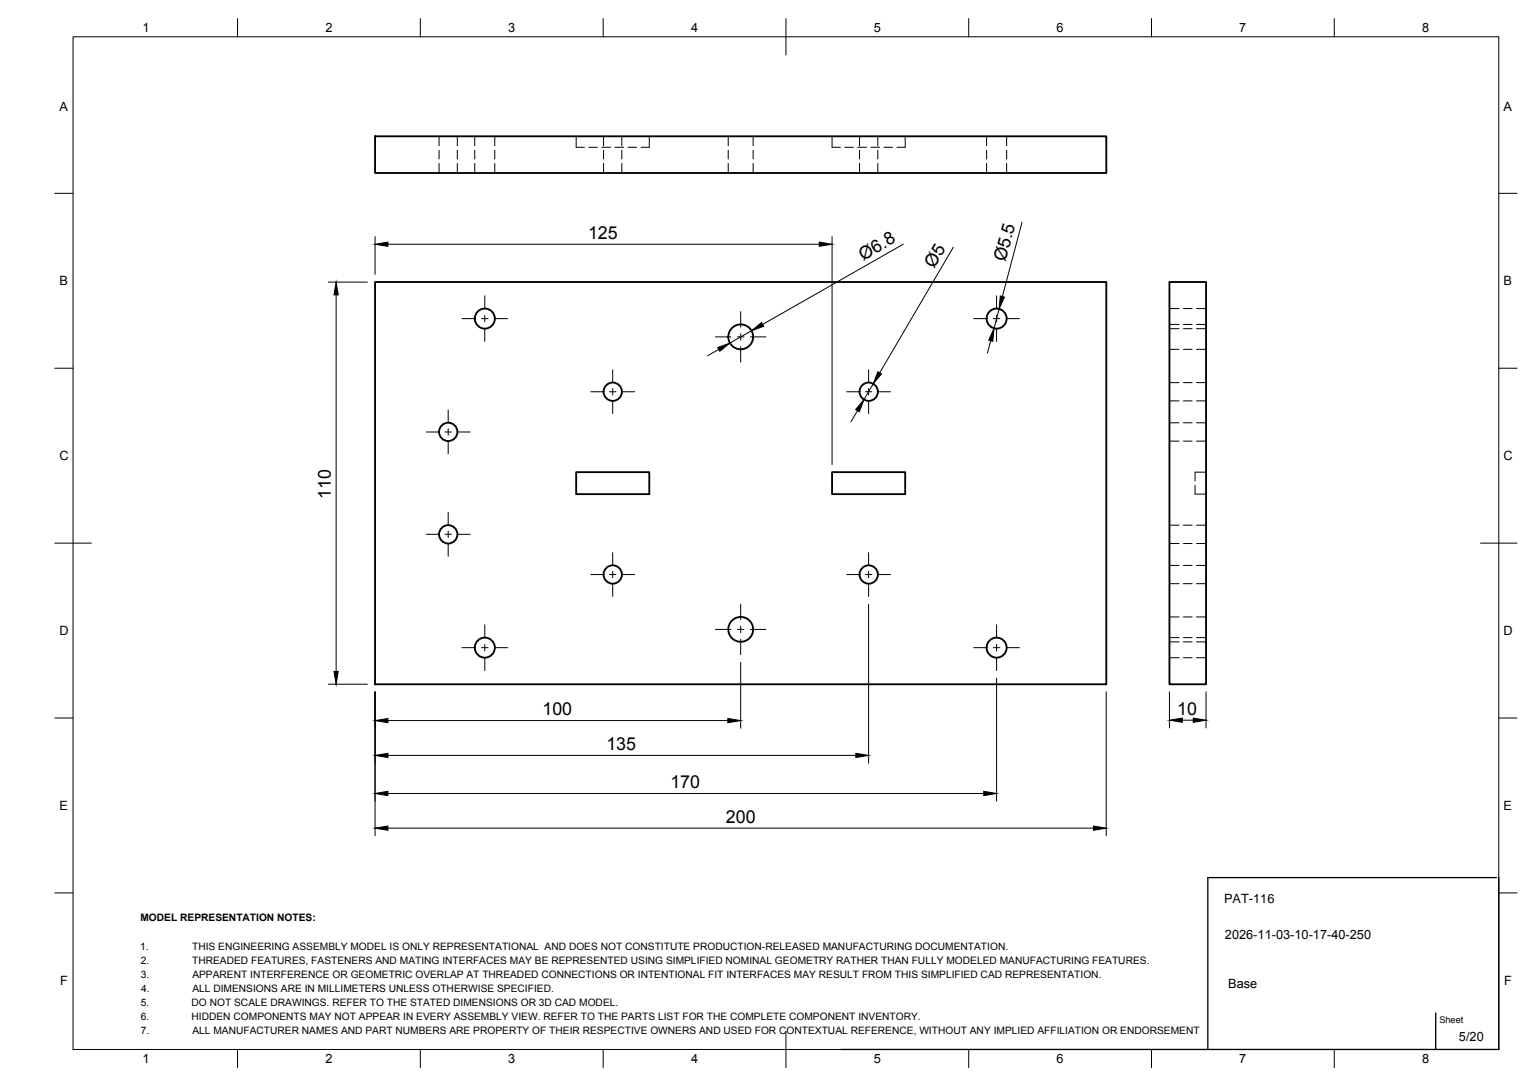
ISO-10303-21;
HEADER;
/* Generated by software containing ST-Developer
 * from STEP Tools, Inc. (www.steptools.com) 
 */

FILE_DESCRIPTION(
/* description */ ('V-block with clamp strap'),
/* implementation_level */ '2;1');

FILE_NAME(
/* name */ 'Base.step',
/* time_stamp */ '2026-10-27T10:50:53-07:00',
/* author */ (''),
/* organization */ (''),
/* preprocessor_version */ 'ST-DEVELOPER v20.2',
/* originating_system */ 'Autodesk Translation Framework v15.17.0.0',
/* authorisation */ '');

FILE_SCHEMA (('AUTOMOTIVE_DESIGN { 1 0 10303 214 3 1 1 }'));
ENDSEC;

DATA;
#10=MECHANICAL_DESIGN_GEOMETRIC_PRESENTATION_REPRESENTATION('',(#266),#7344);
#224=SHAPE_REPRESENTATION_RELATIONSHIP('SRR','None',#7442,#245);
#245=ADVANCED_BREP_SHAPE_REPRESENTATION('',(#287),#7321);
#266=STYLED_ITEM('',(#7610),#287);
#287=MANIFOLD_SOLID_BREP('Body1',#4148);
#305=FACE_BOUND('',#829,.T.);
#306=FACE_BOUND('',#830,.T.);
#307=FACE_BOUND('',#831,.T.);
#308=FACE_BOUND('',#832,.T.);
#309=FACE_BOUND('',#833,.T.);
#310=FACE_BOUND('',#834,.T.);
#311=FACE_BOUND('',#835,.T.);
#312=FACE_BOUND('',#836,.T.);
#313=FACE_BOUND('',#837,.T.);
#314=FACE_BOUND('',#838,.T.);
#315=FACE_BOUND('',#839,.T.);
#316=FACE_BOUND('',#840,.T.);
#317=FACE_BOUND('',#841,.T.);
#318=FACE_BOUND('',#842,.T.);
#319=FACE_BOUND('',#844,.T.);
#320=FACE_BOUND('',#845,.T.);
#321=FACE_BOUND('',#846,.T.);
#322=FACE_BOUND('',#847,.T.);
#323=FACE_BOUND('',#848,.T.);
#324=FACE_BOUND('',#849,.T.);
#325=FACE_BOUND('',#850,.T.);
#326=FACE_BOUND('',#851,.T.);
#327=FACE_BOUND('',#852,.T.);
#328=FACE_BOUND('',#853,.T.);
#329=FACE_BOUND('',#854,.T.);
#330=FACE_BOUND('',#855,.T.);
#376=CIRCLE('',#4418,0.274999999999999);
#377=CIRCLE('',#4419,0.274999999999999);
#378=CIRCLE('',#4421,0.275);
#379=CIRCLE('',#4422,0.275);
#380=CIRCLE('',#4424,0.275);
#381=CIRCLE('',#4425,0.275);
#382=CIRCLE('',#4427,0.274999999999999);
#383=CIRCLE('',#4428,0.274999999999999);
#384=CIRCLE('',#4430,0.34);
#385=CIRCLE('',#4431,0.34);
#386=CIRCLE('',#4433,0.34);
#387=CIRCLE('',#4434,0.34);
#388=CIRCLE('',#4436,0.25);
#389=CIRCLE('',#4437,0.25);
#390=CIRCLE('',#4439,0.25);
#391=CIRCLE('',#4440,0.25);
#392=CIRCLE('',#4442,0.25);
#393=CIRCLE('',#4443,0.25);
#394=CIRCLE('',#4445,0.25);
#395=CIRCLE('',#4446,0.25);
#396=CIRCLE('',#4448,0.25);
#397=CIRCLE('',#4449,0.25);
#398=CIRCLE('',#4451,0.25);
#399=CIRCLE('',#4452,0.25);
#505=CYLINDRICAL_SURFACE('',#4417,0.274999999999999);
#506=CYLINDRICAL_SURFACE('',#4420,0.275);
#507=CYLINDRICAL_SURFACE('',#4423,0.275);
#508=CYLINDRICAL_SURFACE('',#4426,0.274999999999999);
#509=CYLINDRICAL_SURFACE('',#4429,0.34);
#510=CYLINDRICAL_SURFACE('',#4432,0.34);
#511=CYLINDRICAL_SURFACE('',#4435,0.25);
#512=CYLINDRICAL_SURFACE('',#4438,0.25);
#513=CYLINDRICAL_SURFACE('',#4441,0.25);
#514=CYLINDRICAL_SURFACE('',#4444,0.25);
#515=CYLINDRICAL_SURFACE('',#4447,0.25);
#516=CYLINDRICAL_SURFACE('',#4450,0.25);
#562=FACE_OUTER_BOUND('',#802,.T.);
#563=FACE_OUTER_BOUND('',#803,.T.);
#564=FACE_OUTER_BOUND('',#804,.T.);
#565=FACE_OUTER_BOUND('',#805,.T.);
#566=FACE_OUTER_BOUND('',#806,.T.);
#567=FACE_OUTER_BOUND('',#807,.T.);
#568=FACE_OUTER_BOUND('',#808,.T.);
#569=FACE_OUTER_BOUND('',#809,.T.);
#570=FACE_OUTER_BOUND('',#810,.T.);
#571=FACE_OUTER_BOUND('',#811,.T.);
#572=FACE_OUTER_BOUND('',#812,.T.);
#573=FACE_OUTER_BOUND('',#813,.T.);
#574=FACE_OUTER_BOUND('',#814,.T.);
#575=FACE_OUTER_BOUND('',#815,.T.);
#576=FACE_OUTER_BOUND('',#816,.T.);
#577=FACE_OUTER_BOUND('',#817,.T.);
#578=FACE_OUTER_BOUND('',#818,.T.);
#579=FACE_OUTER_BOUND('',#819,.T.);
#580=FACE_OUTER_BOUND('',#820,.T.);
#581=FACE_OUTER_BOUND('',#821,.T.);
#582=FACE_OUTER_BOUND('',#822,.T.);
#583=FACE_OUTER_BOUND('',#823,.T.);
#584=FACE_OUTER_BOUND('',#824,.T.);
#585=FACE_OUTER_BOUND('',#825,.T.);
#586=FACE_OUTER_BOUND('',#826,.T.);
#587=FACE_OUTER_BOUND('',#827,.T.);
#588=FACE_OUTER_BOUND('',#828,.T.);
#589=FACE_OUTER_BOUND('',#843,.T.);
#802=EDGE_LOOP('',(#2696,#2697,#2698,#2699));
#803=EDGE_LOOP('',(#2700,#2701,#2702,#2703));
#804=EDGE_LOOP('',(#2704,#2705,#2706,#2707));
#805=EDGE_LOOP('',(#2708,#2709,#2710,#2711));
#806=EDGE_LOOP('',(#2712,#2713,#2714,#2715));
#807=EDGE_LOOP('',(#2716,#2717,#2718,#2719));
#808=EDGE_LOOP('',(#2720,#2721,#2722,#2723));
#809=EDGE_LOOP('',(#2724,#2725,#2726,#2727));
#810=EDGE_LOOP('',(#2728,#2729,#2730,#2731));
#811=EDGE_LOOP('',(#2732,#2733,#2734,#2735));
#812=EDGE_LOOP('',(#2736,#2737,#2738,#2739));
#813=EDGE_LOOP('',(#2740,#2741,#2742,#2743));
#814=EDGE_LOOP('',(#2744,#2745,#2746,#2747));
#815=EDGE_LOOP('',(#2748,#2749,#2750,#2751));
#816=EDGE_LOOP('',(#2752,#2753,#2754,#2755));
#817=EDGE_LOOP('',(#2756,#2757,#2758,#2759));
#818=EDGE_LOOP('',(#2760,#2761,#2762,#2763));
#819=EDGE_LOOP('',(#2764,#2765,#2766,#2767));
#820=EDGE_LOOP('',(#2768,#2769,#2770,#2771));
#821=EDGE_LOOP('',(#2772,#2773,#2774,#2775));
#822=EDGE_LOOP('',(#2776,#2777,#2778,#2779));
#823=EDGE_LOOP('',(#2780,#2781,#2782,#2783));
#824=EDGE_LOOP('',(#2784,#2785,#2786,#2787));
#825=EDGE_LOOP('',(#2788,#2789,#2790,#2791));
#826=EDGE_LOOP('',(#2792,#2793,#2794,#2795));
#827=EDGE_LOOP('',(#2796,#2797,#2798,#2799));
#828=EDGE_LOOP('',(#2800,#2801,#2802,#2803));
#829=EDGE_LOOP('',(#2804,#2805,#2806,#2807));
#830=EDGE_LOOP('',(#2808));
#831=EDGE_LOOP('',(#2809));
#832=EDGE_LOOP('',(#2810));
#833=EDGE_LOOP('',(#2811));
#834=EDGE_LOOP('',(#2812));
#835=EDGE_LOOP('',(#2813));
#836=EDGE_LOOP('',(#2814));
#837=EDGE_LOOP('',(#2815));
#838=EDGE_LOOP('',(#2816));
#839=EDGE_LOOP('',(#2817));
#840=EDGE_LOOP('',(#2818));
#841=EDGE_LOOP('',(#2819));
#842=EDGE_LOOP('',(#2820,#2821,#2822,#2823));
#843=EDGE_LOOP('',(#2824,#2825,#2826,#2827));
#844=EDGE_LOOP('',(#2828));
#845=EDGE_LOOP('',(#2829));
#846=EDGE_LOOP('',(#2830));
#847=EDGE_LOOP('',(#2831));
#848=EDGE_LOOP('',(#2832));
#849=EDGE_LOOP('',(#2833));
#850=EDGE_LOOP('',(#2834));
#851=EDGE_LOOP('',(#2835));
#852=EDGE_LOOP('',(#2836));
#853=EDGE_LOOP('',(#2837));
#854=EDGE_LOOP('',(#2838));
#855=EDGE_LOOP('',(#2839));
#1113=LINE('',#6092,#1478);
#1114=LINE('',#6094,#1479);
#1115=LINE('',#6096,#1480);
#1116=LINE('',#6097,#1481);
#1117=LINE('',#6100,#1482);
#1118=LINE('',#6102,#1483);
#1119=LINE('',#6103,#1484);
#1120=LINE('',#6106,#1485);
#1121=LINE('',#6108,#1486);
#1122=LINE('',#6109,#1487);
#1123=LINE('',#6111,#1488);
#1124=LINE('',#6112,#1489);
#1125=LINE('',#6117,#1490);
#1126=LINE('',#6119,#1491);
#1127=LINE('',#6121,#1492);
#1128=LINE('',#6122,#1493);
#1129=LINE('',#6125,#1494);
#1130=LINE('',#6127,#1495);
#1131=LINE('',#6128,#1496);
#1132=LINE('',#6131,#1497);
#1133=LINE('',#6133,#1498);
#1134=LINE('',#6134,#1499);
#1135=LINE('',#6136,#1500);
#1136=LINE('',#6137,#1501);
#1137=LINE('',#6143,#1502);
#1138=LINE('',#6149,#1503);
#1139=LINE('',#6155,#1504);
#1140=LINE('',#6161,#1505);
#1141=LINE('',#6167,#1506);
#1142=LINE('',#6173,#1507);
#1143=LINE('',#6179,#1508);
#1144=LINE('',#6185,#1509);
#1145=LINE('',#6191,#1510);
#1146=LINE('',#6197,#1511);
#1147=LINE('',#6203,#1512);
#1148=LINE('',#6209,#1513);
#1149=LINE('',#6214,#1514);
#1150=LINE('',#6216,#1515);
#1151=LINE('',#6218,#1516);
#1152=LINE('',#6219,#1517);
#1153=LINE('',#6222,#1518);
#1154=LINE('',#6224,#1519);
#1155=LINE('',#6225,#1520);
#1156=LINE('',#6228,#1521);
#1157=LINE('',#6230,#1522);
#1158=LINE('',#6231,#1523);
#1159=LINE('',#6233,#1524);
#1160=LINE('',#6234,#1525);
#1478=VECTOR('',#4851,1.);
#1479=VECTOR('',#4852,1.);
#1480=VECTOR('',#4853,1.);
#1481=VECTOR('',#4854,1.);
#1482=VECTOR('',#4857,1.);
#1483=VECTOR('',#4858,1.);
#1484=VECTOR('',#4859,1.);
#1485=VECTOR('',#4862,1.);
#1486=VECTOR('',#4863,1.);
#1487=VECTOR('',#4864,1.);
#1488=VECTOR('',#4867,1.);
#1489=VECTOR('',#4868,1.);
#1490=VECTOR('',#4873,1.);
#1491=VECTOR('',#4874,1.);
#1492=VECTOR('',#4875,1.);
#1493=VECTOR('',#4876,1.);
#1494=VECTOR('',#4879,1.);
#1495=VECTOR('',#4880,1.);
#1496=VECTOR('',#4881,1.);
#1497=VECTOR('',#4884,1.);
#1498=VECTOR('',#4885,1.);
#1499=VECTOR('',#4886,1.);
#1500=VECTOR('',#4889,1.);
#1501=VECTOR('',#4890,1.);
#1502=VECTOR('',#4897,0.274999999999999);
#1503=VECTOR('',#4904,0.275);
#1504=VECTOR('',#4911,0.275);
#1505=VECTOR('',#4918,0.274999999999999);
#1506=VECTOR('',#4925,0.34);
#1507=VECTOR('',#4932,0.34);
#1508=VECTOR('',#4939,0.25);
#1509=VECTOR('',#4946,0.25);
#1510=VECTOR('',#4953,0.25);
#1511=VECTOR('',#4960,0.25);
#1512=VECTOR('',#4967,0.25);
#1513=VECTOR('',#4974,0.25);
#1514=VECTOR('',#4979,1.);
#1515=VECTOR('',#4980,1.);
#1516=VECTOR('',#4981,1.);
#1517=VECTOR('',#4982,1.);
#1518=VECTOR('',#4985,1.);
#1519=VECTOR('',#4986,1.);
#1520=VECTOR('',#4987,1.);
#1521=VECTOR('',#4990,1.);
#1522=VECTOR('',#4991,1.);
#1523=VECTOR('',#4992,1.);
#1524=VECTOR('',#4995,1.);
#1525=VECTOR('',#4996,1.);
#1843=VERTEX_POINT('',#6090);
#1844=VERTEX_POINT('',#6091);
#1845=VERTEX_POINT('',#6093);
#1846=VERTEX_POINT('',#6095);
#1847=VERTEX_POINT('',#6099);
#1848=VERTEX_POINT('',#6101);
#1849=VERTEX_POINT('',#6105);
#1850=VERTEX_POINT('',#6107);
#1851=VERTEX_POINT('',#6115);
#1852=VERTEX_POINT('',#6116);
#1853=VERTEX_POINT('',#6118);
#1854=VERTEX_POINT('',#6120);
#1855=VERTEX_POINT('',#6124);
#1856=VERTEX_POINT('',#6126);
#1857=VERTEX_POINT('',#6130);
#1858=VERTEX_POINT('',#6132);
#1859=VERTEX_POINT('',#6140);
#1860=VERTEX_POINT('',#6142);
#1861=VERTEX_POINT('',#6146);
#1862=VERTEX_POINT('',#6148);
#1863=VERTEX_POINT('',#6152);
#1864=VERTEX_POINT('',#6154);
#1865=VERTEX_POINT('',#6158);
#1866=VERTEX_POINT('',#6160);
#1867=VERTEX_POINT('',#6164);
#1868=VERTEX_POINT('',#6166);
#1869=VERTEX_POINT('',#6170);
#1870=VERTEX_POINT('',#6172);
#1871=VERTEX_POINT('',#6176);
#1872=VERTEX_POINT('',#6178);
#1873=VERTEX_POINT('',#6182);
#1874=VERTEX_POINT('',#6184);
#1875=VERTEX_POINT('',#6188);
#1876=VERTEX_POINT('',#6190);
#1877=VERTEX_POINT('',#6194);
#1878=VERTEX_POINT('',#6196);
#1879=VERTEX_POINT('',#6200);
#1880=VERTEX_POINT('',#6202);
#1881=VERTEX_POINT('',#6206);
#1882=VERTEX_POINT('',#6208);
#1883=VERTEX_POINT('',#6212);
#1884=VERTEX_POINT('',#6213);
#1885=VERTEX_POINT('',#6215);
#1886=VERTEX_POINT('',#6217);
#1887=VERTEX_POINT('',#6221);
#1888=VERTEX_POINT('',#6223);
#1889=VERTEX_POINT('',#6227);
#1890=VERTEX_POINT('',#6229);
#2174=EDGE_CURVE('',#1843,#1844,#1113,.T.);
#2175=EDGE_CURVE('',#1845,#1843,#1114,.T.);
#2176=EDGE_CURVE('',#1846,#1845,#1115,.T.);
#2177=EDGE_CURVE('',#1846,#1844,#1116,.T.);
#2178=EDGE_CURVE('',#1844,#1847,#1117,.T.);
#2179=EDGE_CURVE('',#1848,#1846,#1118,.T.);
#2180=EDGE_CURVE('',#1848,#1847,#1119,.T.);
#2181=EDGE_CURVE('',#1847,#1849,#1120,.T.);
#2182=EDGE_CURVE('',#1850,#1848,#1121,.T.);
#2183=EDGE_CURVE('',#1850,#1849,#1122,.T.);
#2184=EDGE_CURVE('',#1849,#1843,#1123,.T.);
#2185=EDGE_CURVE('',#1845,#1850,#1124,.T.);
#2186=EDGE_CURVE('',#1851,#1852,#1125,.T.);
#2187=EDGE_CURVE('',#1853,#1851,#1126,.T.);
#2188=EDGE_CURVE('',#1854,#1853,#1127,.T.);
#2189=EDGE_CURVE('',#1854,#1852,#1128,.T.);
#2190=EDGE_CURVE('',#1852,#1855,#1129,.T.);
#2191=EDGE_CURVE('',#1856,#1854,#1130,.T.);
#2192=EDGE_CURVE('',#1856,#1855,#1131,.T.);
#2193=EDGE_CURVE('',#1855,#1857,#1132,.T.);
#2194=EDGE_CURVE('',#1858,#1856,#1133,.T.);
#2195=EDGE_CURVE('',#1858,#1857,#1134,.T.);
#2196=EDGE_CURVE('',#1857,#1851,#1135,.T.);
#2197=EDGE_CURVE('',#1853,#1858,#1136,.T.);
#2198=EDGE_CURVE('',#1859,#1859,#376,.T.);
#2199=EDGE_CURVE('',#1859,#1860,#1137,.T.);
#2200=EDGE_CURVE('',#1860,#1860,#377,.T.);
#2201=EDGE_CURVE('',#1861,#1861,#378,.T.);
#2202=EDGE_CURVE('',#1861,#1862,#1138,.T.);
#2203=EDGE_CURVE('',#1862,#1862,#379,.T.);
#2204=EDGE_CURVE('',#1863,#1863,#380,.T.);
#2205=EDGE_CURVE('',#1863,#1864,#1139,.T.);
#2206=EDGE_CURVE('',#1864,#1864,#381,.T.);
#2207=EDGE_CURVE('',#1865,#1865,#382,.T.);
#2208=EDGE_CURVE('',#1865,#1866,#1140,.T.);
#2209=EDGE_CURVE('',#1866,#1866,#383,.T.);
#2210=EDGE_CURVE('',#1867,#1867,#384,.T.);
#2211=EDGE_CURVE('',#1867,#1868,#1141,.T.);
#2212=EDGE_CURVE('',#1868,#1868,#385,.T.);
#2213=EDGE_CURVE('',#1869,#1869,#386,.T.);
#2214=EDGE_CURVE('',#1869,#1870,#1142,.T.);
#2215=EDGE_CURVE('',#1870,#1870,#387,.T.);
#2216=EDGE_CURVE('',#1871,#1871,#388,.T.);
#2217=EDGE_CURVE('',#1871,#1872,#1143,.T.);
#2218=EDGE_CURVE('',#1872,#1872,#389,.T.);
#2219=EDGE_CURVE('',#1873,#1873,#390,.T.);
#2220=EDGE_CURVE('',#1873,#1874,#1144,.T.);
#2221=EDGE_CURVE('',#1874,#1874,#391,.T.);
#2222=EDGE_CURVE('',#1875,#1875,#392,.T.);
#2223=EDGE_CURVE('',#1875,#1876,#1145,.T.);
#2224=EDGE_CURVE('',#1876,#1876,#393,.T.);
#2225=EDGE_CURVE('',#1877,#1877,#394,.T.);
#2226=EDGE_CURVE('',#1877,#1878,#1146,.T.);
#2227=EDGE_CURVE('',#1878,#1878,#395,.T.);
#2228=EDGE_CURVE('',#1879,#1879,#396,.T.);
#2229=EDGE_CURVE('',#1879,#1880,#1147,.T.);
#2230=EDGE_CURVE('',#1880,#1880,#397,.T.);
#2231=EDGE_CURVE('',#1881,#1881,#398,.T.);
#2232=EDGE_CURVE('',#1881,#1882,#1148,.T.);
#2233=EDGE_CURVE('',#1882,#1882,#399,.T.);
#2234=EDGE_CURVE('',#1883,#1884,#1149,.T.);
#2235=EDGE_CURVE('',#1884,#1885,#1150,.T.);
#2236=EDGE_CURVE('',#1886,#1885,#1151,.T.);
#2237=EDGE_CURVE('',#1883,#1886,#1152,.T.);
#2238=EDGE_CURVE('',#1887,#1883,#1153,.T.);
#2239=EDGE_CURVE('',#1888,#1886,#1154,.T.);
#2240=EDGE_CURVE('',#1887,#1888,#1155,.T.);
#2241=EDGE_CURVE('',#1889,#1887,#1156,.T.);
#2242=EDGE_CURVE('',#1890,#1888,#1157,.T.);
#2243=EDGE_CURVE('',#1889,#1890,#1158,.T.);
#2244=EDGE_CURVE('',#1884,#1889,#1159,.T.);
#2245=EDGE_CURVE('',#1885,#1890,#1160,.T.);
#2696=ORIENTED_EDGE('',*,*,#2174,.F.);
#2697=ORIENTED_EDGE('',*,*,#2175,.F.);
#2698=ORIENTED_EDGE('',*,*,#2176,.F.);
#2699=ORIENTED_EDGE('',*,*,#2177,.T.);
#2700=ORIENTED_EDGE('',*,*,#2178,.F.);
#2701=ORIENTED_EDGE('',*,*,#2177,.F.);
#2702=ORIENTED_EDGE('',*,*,#2179,.F.);
#2703=ORIENTED_EDGE('',*,*,#2180,.T.);
#2704=ORIENTED_EDGE('',*,*,#2181,.F.);
#2705=ORIENTED_EDGE('',*,*,#2180,.F.);
#2706=ORIENTED_EDGE('',*,*,#2182,.F.);
#2707=ORIENTED_EDGE('',*,*,#2183,.T.);
#2708=ORIENTED_EDGE('',*,*,#2184,.F.);
#2709=ORIENTED_EDGE('',*,*,#2183,.F.);
#2710=ORIENTED_EDGE('',*,*,#2185,.F.);
#2711=ORIENTED_EDGE('',*,*,#2175,.T.);
#2712=ORIENTED_EDGE('',*,*,#2179,.T.);
#2713=ORIENTED_EDGE('',*,*,#2176,.T.);
#2714=ORIENTED_EDGE('',*,*,#2185,.T.);
#2715=ORIENTED_EDGE('',*,*,#2182,.T.);
#2716=ORIENTED_EDGE('',*,*,#2186,.F.);
#2717=ORIENTED_EDGE('',*,*,#2187,.F.);
#2718=ORIENTED_EDGE('',*,*,#2188,.F.);
#2719=ORIENTED_EDGE('',*,*,#2189,.T.);
#2720=ORIENTED_EDGE('',*,*,#2190,.F.);
#2721=ORIENTED_EDGE('',*,*,#2189,.F.);
#2722=ORIENTED_EDGE('',*,*,#2191,.F.);
#2723=ORIENTED_EDGE('',*,*,#2192,.T.);
#2724=ORIENTED_EDGE('',*,*,#2193,.F.);
#2725=ORIENTED_EDGE('',*,*,#2192,.F.);
#2726=ORIENTED_EDGE('',*,*,#2194,.F.);
#2727=ORIENTED_EDGE('',*,*,#2195,.T.);
#2728=ORIENTED_EDGE('',*,*,#2196,.F.);
#2729=ORIENTED_EDGE('',*,*,#2195,.F.);
#2730=ORIENTED_EDGE('',*,*,#2197,.F.);
#2731=ORIENTED_EDGE('',*,*,#2187,.T.);
#2732=ORIENTED_EDGE('',*,*,#2191,.T.);
#2733=ORIENTED_EDGE('',*,*,#2188,.T.);
#2734=ORIENTED_EDGE('',*,*,#2197,.T.);
#2735=ORIENTED_EDGE('',*,*,#2194,.T.);
#2736=ORIENTED_EDGE('',*,*,#2198,.F.);
#2737=ORIENTED_EDGE('',*,*,#2199,.T.);
#2738=ORIENTED_EDGE('',*,*,#2200,.F.);
#2739=ORIENTED_EDGE('',*,*,#2199,.F.);
#2740=ORIENTED_EDGE('',*,*,#2201,.F.);
#2741=ORIENTED_EDGE('',*,*,#2202,.T.);
#2742=ORIENTED_EDGE('',*,*,#2203,.F.);
#2743=ORIENTED_EDGE('',*,*,#2202,.F.);
#2744=ORIENTED_EDGE('',*,*,#2204,.F.);
#2745=ORIENTED_EDGE('',*,*,#2205,.T.);
#2746=ORIENTED_EDGE('',*,*,#2206,.F.);
#2747=ORIENTED_EDGE('',*,*,#2205,.F.);
#2748=ORIENTED_EDGE('',*,*,#2207,.F.);
#2749=ORIENTED_EDGE('',*,*,#2208,.T.);
#2750=ORIENTED_EDGE('',*,*,#2209,.F.);
#2751=ORIENTED_EDGE('',*,*,#2208,.F.);
#2752=ORIENTED_EDGE('',*,*,#2210,.F.);
#2753=ORIENTED_EDGE('',*,*,#2211,.T.);
#2754=ORIENTED_EDGE('',*,*,#2212,.F.);
#2755=ORIENTED_EDGE('',*,*,#2211,.F.);
#2756=ORIENTED_EDGE('',*,*,#2213,.F.);
#2757=ORIENTED_EDGE('',*,*,#2214,.T.);
#2758=ORIENTED_EDGE('',*,*,#2215,.F.);
#2759=ORIENTED_EDGE('',*,*,#2214,.F.);
#2760=ORIENTED_EDGE('',*,*,#2216,.F.);
#2761=ORIENTED_EDGE('',*,*,#2217,.T.);
#2762=ORIENTED_EDGE('',*,*,#2218,.F.);
#2763=ORIENTED_EDGE('',*,*,#2217,.F.);
#2764=ORIENTED_EDGE('',*,*,#2219,.F.);
#2765=ORIENTED_EDGE('',*,*,#2220,.T.);
#2766=ORIENTED_EDGE('',*,*,#2221,.F.);
#2767=ORIENTED_EDGE('',*,*,#2220,.F.);
#2768=ORIENTED_EDGE('',*,*,#2222,.F.);
#2769=ORIENTED_EDGE('',*,*,#2223,.T.);
#2770=ORIENTED_EDGE('',*,*,#2224,.F.);
#2771=ORIENTED_EDGE('',*,*,#2223,.F.);
#2772=ORIENTED_EDGE('',*,*,#2225,.F.);
#2773=ORIENTED_EDGE('',*,*,#2226,.T.);
#2774=ORIENTED_EDGE('',*,*,#2227,.F.);
#2775=ORIENTED_EDGE('',*,*,#2226,.F.);
#2776=ORIENTED_EDGE('',*,*,#2228,.F.);
#2777=ORIENTED_EDGE('',*,*,#2229,.T.);
#2778=ORIENTED_EDGE('',*,*,#2230,.F.);
#2779=ORIENTED_EDGE('',*,*,#2229,.F.);
#2780=ORIENTED_EDGE('',*,*,#2231,.F.);
#2781=ORIENTED_EDGE('',*,*,#2232,.T.);
#2782=ORIENTED_EDGE('',*,*,#2233,.F.);
#2783=ORIENTED_EDGE('',*,*,#2232,.F.);
#2784=ORIENTED_EDGE('',*,*,#2234,.T.);
#2785=ORIENTED_EDGE('',*,*,#2235,.T.);
#2786=ORIENTED_EDGE('',*,*,#2236,.F.);
#2787=ORIENTED_EDGE('',*,*,#2237,.F.);
#2788=ORIENTED_EDGE('',*,*,#2238,.T.);
#2789=ORIENTED_EDGE('',*,*,#2237,.T.);
#2790=ORIENTED_EDGE('',*,*,#2239,.F.);
#2791=ORIENTED_EDGE('',*,*,#2240,.F.);
#2792=ORIENTED_EDGE('',*,*,#2241,.T.);
#2793=ORIENTED_EDGE('',*,*,#2240,.T.);
#2794=ORIENTED_EDGE('',*,*,#2242,.F.);
#2795=ORIENTED_EDGE('',*,*,#2243,.F.);
#2796=ORIENTED_EDGE('',*,*,#2244,.T.);
#2797=ORIENTED_EDGE('',*,*,#2243,.T.);
#2798=ORIENTED_EDGE('',*,*,#2245,.F.);
#2799=ORIENTED_EDGE('',*,*,#2235,.F.);
#2800=ORIENTED_EDGE('',*,*,#2245,.T.);
#2801=ORIENTED_EDGE('',*,*,#2242,.T.);
#2802=ORIENTED_EDGE('',*,*,#2239,.T.);
#2803=ORIENTED_EDGE('',*,*,#2236,.T.);
#2804=ORIENTED_EDGE('',*,*,#2193,.T.);
#2805=ORIENTED_EDGE('',*,*,#2196,.T.);
#2806=ORIENTED_EDGE('',*,*,#2186,.T.);
#2807=ORIENTED_EDGE('',*,*,#2190,.T.);
#2808=ORIENTED_EDGE('',*,*,#2212,.T.);
#2809=ORIENTED_EDGE('',*,*,#2215,.T.);
#2810=ORIENTED_EDGE('',*,*,#2233,.T.);
#2811=ORIENTED_EDGE('',*,*,#2230,.T.);
#2812=ORIENTED_EDGE('',*,*,#2227,.T.);
#2813=ORIENTED_EDGE('',*,*,#2224,.T.);
#2814=ORIENTED_EDGE('',*,*,#2221,.T.);
#2815=ORIENTED_EDGE('',*,*,#2218,.T.);
#2816=ORIENTED_EDGE('',*,*,#2209,.T.);
#2817=ORIENTED_EDGE('',*,*,#2206,.T.);
#2818=ORIENTED_EDGE('',*,*,#2203,.T.);
#2819=ORIENTED_EDGE('',*,*,#2200,.T.);
#2820=ORIENTED_EDGE('',*,*,#2181,.T.);
#2821=ORIENTED_EDGE('',*,*,#2184,.T.);
#2822=ORIENTED_EDGE('',*,*,#2174,.T.);
#2823=ORIENTED_EDGE('',*,*,#2178,.T.);
#2824=ORIENTED_EDGE('',*,*,#2244,.F.);
#2825=ORIENTED_EDGE('',*,*,#2234,.F.);
#2826=ORIENTED_EDGE('',*,*,#2238,.F.);
#2827=ORIENTED_EDGE('',*,*,#2241,.F.);
#2828=ORIENTED_EDGE('',*,*,#2210,.T.);
#2829=ORIENTED_EDGE('',*,*,#2213,.T.);
#2830=ORIENTED_EDGE('',*,*,#2231,.T.);
#2831=ORIENTED_EDGE('',*,*,#2228,.T.);
#2832=ORIENTED_EDGE('',*,*,#2225,.T.);
#2833=ORIENTED_EDGE('',*,*,#2222,.T.);
#2834=ORIENTED_EDGE('',*,*,#2219,.T.);
#2835=ORIENTED_EDGE('',*,*,#2216,.T.);
#2836=ORIENTED_EDGE('',*,*,#2207,.T.);
#2837=ORIENTED_EDGE('',*,*,#2204,.T.);
#2838=ORIENTED_EDGE('',*,*,#2201,.T.);
#2839=ORIENTED_EDGE('',*,*,#2198,.T.);
#3740=PLANE('',#4407);
#3741=PLANE('',#4408);
#3742=PLANE('',#4409);
#3743=PLANE('',#4410);
#3744=PLANE('',#4411);
#3745=PLANE('',#4412);
#3746=PLANE('',#4413);
#3747=PLANE('',#4414);
#3748=PLANE('',#4415);
#3749=PLANE('',#4416);
#3750=PLANE('',#4453);
#3751=PLANE('',#4454);
#3752=PLANE('',#4455);
#3753=PLANE('',#4456);
#3754=PLANE('',#4457);
#3755=PLANE('',#4458);
#3908=ADVANCED_FACE('',(#562),#3740,.F.);
#3909=ADVANCED_FACE('',(#563),#3741,.F.);
#3910=ADVANCED_FACE('',(#564),#3742,.F.);
#3911=ADVANCED_FACE('',(#565),#3743,.F.);
#3912=ADVANCED_FACE('',(#566),#3744,.T.);
#3913=ADVANCED_FACE('',(#567),#3745,.F.);
#3914=ADVANCED_FACE('',(#568),#3746,.F.);
#3915=ADVANCED_FACE('',(#569),#3747,.F.);
#3916=ADVANCED_FACE('',(#570),#3748,.F.);
#3917=ADVANCED_FACE('',(#571),#3749,.T.);
#3918=ADVANCED_FACE('',(#572),#505,.F.);
#3919=ADVANCED_FACE('',(#573),#506,.F.);
#3920=ADVANCED_FACE('',(#574),#507,.F.);
#3921=ADVANCED_FACE('',(#575),#508,.F.);
#3922=ADVANCED_FACE('',(#576),#509,.F.);
#3923=ADVANCED_FACE('',(#577),#510,.F.);
#3924=ADVANCED_FACE('',(#578),#511,.F.);
#3925=ADVANCED_FACE('',(#579),#512,.F.);
#3926=ADVANCED_FACE('',(#580),#513,.F.);
#3927=ADVANCED_FACE('',(#581),#514,.F.);
#3928=ADVANCED_FACE('',(#582),#515,.F.);
#3929=ADVANCED_FACE('',(#583),#516,.F.);
#3930=ADVANCED_FACE('',(#584),#3750,.T.);
#3931=ADVANCED_FACE('',(#585),#3751,.T.);
#3932=ADVANCED_FACE('',(#586),#3752,.T.);
#3933=ADVANCED_FACE('',(#587),#3753,.T.);
#3934=ADVANCED_FACE('',(#588,#305,#306,#307,#308,#309,#310,#311,#312,#313,
#314,#315,#316,#317,#318),#3754,.T.);
#3935=ADVANCED_FACE('',(#589,#319,#320,#321,#322,#323,#324,#325,#326,#327,
#328,#329,#330),#3755,.F.);
#4148=CLOSED_SHELL('',(#3908,#3909,#3910,#3911,#3912,#3913,#3914,#3915,
#3916,#3917,#3918,#3919,#3920,#3921,#3922,#3923,#3924,#3925,#3926,#3927,
#3928,#3929,#3930,#3931,#3932,#3933,#3934,#3935));
#4406=AXIS2_PLACEMENT_3D('',#6088,#4847,#4848);
#4407=AXIS2_PLACEMENT_3D('',#6089,#4849,#4850);
#4408=AXIS2_PLACEMENT_3D('',#6098,#4855,#4856);
#4409=AXIS2_PLACEMENT_3D('',#6104,#4860,#4861);
#4410=AXIS2_PLACEMENT_3D('',#6110,#4865,#4866);
#4411=AXIS2_PLACEMENT_3D('',#6113,#4869,#4870);
#4412=AXIS2_PLACEMENT_3D('',#6114,#4871,#4872);
#4413=AXIS2_PLACEMENT_3D('',#6123,#4877,#4878);
#4414=AXIS2_PLACEMENT_3D('',#6129,#4882,#4883);
#4415=AXIS2_PLACEMENT_3D('',#6135,#4887,#4888);
#4416=AXIS2_PLACEMENT_3D('',#6138,#4891,#4892);
#4417=AXIS2_PLACEMENT_3D('',#6139,#4893,#4894);
#4418=AXIS2_PLACEMENT_3D('',#6141,#4895,#4896);
#4419=AXIS2_PLACEMENT_3D('',#6144,#4898,#4899);
#4420=AXIS2_PLACEMENT_3D('',#6145,#4900,#4901);
#4421=AXIS2_PLACEMENT_3D('',#6147,#4902,#4903);
#4422=AXIS2_PLACEMENT_3D('',#6150,#4905,#4906);
#4423=AXIS2_PLACEMENT_3D('',#6151,#4907,#4908);
#4424=AXIS2_PLACEMENT_3D('',#6153,#4909,#4910);
#4425=AXIS2_PLACEMENT_3D('',#6156,#4912,#4913);
#4426=AXIS2_PLACEMENT_3D('',#6157,#4914,#4915);
#4427=AXIS2_PLACEMENT_3D('',#6159,#4916,#4917);
#4428=AXIS2_PLACEMENT_3D('',#6162,#4919,#4920);
#4429=AXIS2_PLACEMENT_3D('',#6163,#4921,#4922);
#4430=AXIS2_PLACEMENT_3D('',#6165,#4923,#4924);
#4431=AXIS2_PLACEMENT_3D('',#6168,#4926,#4927);
#4432=AXIS2_PLACEMENT_3D('',#6169,#4928,#4929);
#4433=AXIS2_PLACEMENT_3D('',#6171,#4930,#4931);
#4434=AXIS2_PLACEMENT_3D('',#6174,#4933,#4934);
#4435=AXIS2_PLACEMENT_3D('',#6175,#4935,#4936);
#4436=AXIS2_PLACEMENT_3D('',#6177,#4937,#4938);
#4437=AXIS2_PLACEMENT_3D('',#6180,#4940,#4941);
#4438=AXIS2_PLACEMENT_3D('',#6181,#4942,#4943);
#4439=AXIS2_PLACEMENT_3D('',#6183,#4944,#4945);
#4440=AXIS2_PLACEMENT_3D('',#6186,#4947,#4948);
#4441=AXIS2_PLACEMENT_3D('',#6187,#4949,#4950);
#4442=AXIS2_PLACEMENT_3D('',#6189,#4951,#4952);
#4443=AXIS2_PLACEMENT_3D('',#6192,#4954,#4955);
#4444=AXIS2_PLACEMENT_3D('',#6193,#4956,#4957);
#4445=AXIS2_PLACEMENT_3D('',#6195,#4958,#4959);
#4446=AXIS2_PLACEMENT_3D('',#6198,#4961,#4962);
#4447=AXIS2_PLACEMENT_3D('',#6199,#4963,#4964);
#4448=AXIS2_PLACEMENT_3D('',#6201,#4965,#4966);
#4449=AXIS2_PLACEMENT_3D('',#6204,#4968,#4969);
#4450=AXIS2_PLACEMENT_3D('',#6205,#4970,#4971);
#4451=AXIS2_PLACEMENT_3D('',#6207,#4972,#4973);
#4452=AXIS2_PLACEMENT_3D('',#6210,#4975,#4976);
#4453=AXIS2_PLACEMENT_3D('',#6211,#4977,#4978);
#4454=AXIS2_PLACEMENT_3D('',#6220,#4983,#4984);
#4455=AXIS2_PLACEMENT_3D('',#6226,#4988,#4989);
#4456=AXIS2_PLACEMENT_3D('',#6232,#4993,#4994);
#4457=AXIS2_PLACEMENT_3D('',#6235,#4997,#4998);
#4458=AXIS2_PLACEMENT_3D('',#6236,#4999,#5000);
#4847=DIRECTION('axis',(0.,0.,1.));
#4848=DIRECTION('refdir',(1.,0.,0.));
#4849=DIRECTION('center_axis',(0.,-1.,0.));
#4850=DIRECTION('ref_axis',(1.,0.,0.));
#4851=DIRECTION('',(-1.,0.,0.));
#4852=DIRECTION('',(0.,0.,1.));
#4853=DIRECTION('',(1.,0.,0.));
#4854=DIRECTION('',(0.,0.,1.));
#4855=DIRECTION('center_axis',(-1.,0.,0.));
#4856=DIRECTION('ref_axis',(0.,-1.,0.));
#4857=DIRECTION('',(0.,1.,0.));
#4858=DIRECTION('',(0.,-1.,0.));
#4859=DIRECTION('',(0.,0.,1.));
#4860=DIRECTION('center_axis',(0.,1.,0.));
#4861=DIRECTION('ref_axis',(-1.,0.,0.));
#4862=DIRECTION('',(1.,0.,0.));
#4863=DIRECTION('',(-1.,0.,0.));
#4864=DIRECTION('',(0.,0.,1.));
#4865=DIRECTION('center_axis',(1.,0.,0.));
#4866=DIRECTION('ref_axis',(0.,1.,0.));
#4867=DIRECTION('',(0.,-1.,0.));
#4868=DIRECTION('',(0.,1.,0.));
#4869=DIRECTION('center_axis',(0.,0.,1.));
#4870=DIRECTION('ref_axis',(1.,0.,0.));
#4871=DIRECTION('center_axis',(0.,-1.,0.));
#4872=DIRECTION('ref_axis',(1.,0.,0.));
#4873=DIRECTION('',(-1.,0.,0.));
#4874=DIRECTION('',(0.,0.,1.));
#4875=DIRECTION('',(1.,0.,0.));
#4876=DIRECTION('',(0.,0.,1.));
#4877=DIRECTION('center_axis',(-1.,0.,0.));
#4878=DIRECTION('ref_axis',(0.,-1.,0.));
#4879=DIRECTION('',(0.,1.,0.));
#4880=DIRECTION('',(0.,-1.,0.));
#4881=DIRECTION('',(0.,0.,1.));
#4882=DIRECTION('center_axis',(0.,1.,0.));
#4883=DIRECTION('ref_axis',(-1.,0.,0.));
#4884=DIRECTION('',(1.,0.,0.));
#4885=DIRECTION('',(-1.,0.,0.));
#4886=DIRECTION('',(0.,0.,1.));
#4887=DIRECTION('center_axis',(1.,0.,0.));
#4888=DIRECTION('ref_axis',(0.,1.,0.));
#4889=DIRECTION('',(0.,-1.,0.));
#4890=DIRECTION('',(0.,1.,0.));
#4891=DIRECTION('center_axis',(0.,0.,1.));
#4892=DIRECTION('ref_axis',(1.,0.,0.));
#4893=DIRECTION('center_axis',(0.,0.,1.));
#4894=DIRECTION('ref_axis',(1.,0.,0.));
#4895=DIRECTION('center_axis',(0.,0.,1.));
#4896=DIRECTION('ref_axis',(1.,0.,0.));
#4897=DIRECTION('',(0.,0.,1.));
#4898=DIRECTION('center_axis',(0.,0.,-1.));
#4899=DIRECTION('ref_axis',(1.,0.,0.));
#4900=DIRECTION('center_axis',(0.,0.,1.));
#4901=DIRECTION('ref_axis',(1.,0.,0.));
#4902=DIRECTION('center_axis',(0.,0.,1.));
#4903=DIRECTION('ref_axis',(1.,0.,0.));
#4904=DIRECTION('',(0.,0.,1.));
#4905=DIRECTION('center_axis',(0.,0.,-1.));
#4906=DIRECTION('ref_axis',(1.,0.,0.));
#4907=DIRECTION('center_axis',(0.,0.,1.));
#4908=DIRECTION('ref_axis',(1.,0.,0.));
#4909=DIRECTION('center_axis',(0.,0.,1.));
#4910=DIRECTION('ref_axis',(1.,0.,0.));
#4911=DIRECTION('',(0.,0.,1.));
#4912=DIRECTION('center_axis',(0.,0.,-1.));
#4913=DIRECTION('ref_axis',(1.,0.,0.));
#4914=DIRECTION('center_axis',(0.,0.,1.));
#4915=DIRECTION('ref_axis',(1.,0.,0.));
#4916=DIRECTION('center_axis',(0.,0.,1.));
#4917=DIRECTION('ref_axis',(1.,0.,0.));
#4918=DIRECTION('',(0.,0.,1.));
#4919=DIRECTION('center_axis',(0.,0.,-1.));
#4920=DIRECTION('ref_axis',(1.,0.,0.));
#4921=DIRECTION('center_axis',(0.,0.,1.));
#4922=DIRECTION('ref_axis',(1.,0.,0.));
#4923=DIRECTION('center_axis',(0.,0.,1.));
#4924=DIRECTION('ref_axis',(1.,0.,0.));
#4925=DIRECTION('',(0.,0.,1.));
#4926=DIRECTION('center_axis',(0.,0.,-1.));
#4927=DIRECTION('ref_axis',(1.,0.,0.));
#4928=DIRECTION('center_axis',(0.,0.,1.));
#4929=DIRECTION('ref_axis',(1.,0.,0.));
#4930=DIRECTION('center_axis',(0.,0.,1.));
#4931=DIRECTION('ref_axis',(1.,0.,0.));
#4932=DIRECTION('',(0.,0.,1.));
#4933=DIRECTION('center_axis',(0.,0.,-1.));
#4934=DIRECTION('ref_axis',(1.,0.,0.));
#4935=DIRECTION('center_axis',(0.,0.,1.));
#4936=DIRECTION('ref_axis',(1.,0.,0.));
#4937=DIRECTION('center_axis',(0.,0.,1.));
#4938=DIRECTION('ref_axis',(1.,0.,0.));
#4939=DIRECTION('',(0.,0.,1.));
#4940=DIRECTION('center_axis',(0.,0.,-1.));
#4941=DIRECTION('ref_axis',(1.,0.,0.));
#4942=DIRECTION('center_axis',(0.,0.,1.));
#4943=DIRECTION('ref_axis',(1.,0.,0.));
#4944=DIRECTION('center_axis',(0.,0.,1.));
#4945=DIRECTION('ref_axis',(1.,0.,0.));
#4946=DIRECTION('',(0.,0.,1.));
#4947=DIRECTION('center_axis',(0.,0.,-1.));
#4948=DIRECTION('ref_axis',(1.,0.,0.));
#4949=DIRECTION('center_axis',(0.,0.,1.));
#4950=DIRECTION('ref_axis',(1.,0.,0.));
#4951=DIRECTION('center_axis',(0.,0.,1.));
#4952=DIRECTION('ref_axis',(1.,0.,0.));
#4953=DIRECTION('',(0.,0.,1.));
#4954=DIRECTION('center_axis',(0.,0.,-1.));
#4955=DIRECTION('ref_axis',(1.,0.,0.));
#4956=DIRECTION('center_axis',(0.,0.,1.));
#4957=DIRECTION('ref_axis',(1.,0.,0.));
#4958=DIRECTION('center_axis',(0.,0.,1.));
#4959=DIRECTION('ref_axis',(1.,0.,0.));
#4960=DIRECTION('',(0.,0.,1.));
#4961=DIRECTION('center_axis',(0.,0.,-1.));
#4962=DIRECTION('ref_axis',(1.,0.,0.));
#4963=DIRECTION('center_axis',(0.,0.,1.));
#4964=DIRECTION('ref_axis',(1.,0.,0.));
#4965=DIRECTION('center_axis',(0.,0.,1.));
#4966=DIRECTION('ref_axis',(1.,0.,0.));
#4967=DIRECTION('',(0.,0.,1.));
#4968=DIRECTION('center_axis',(0.,0.,-1.));
#4969=DIRECTION('ref_axis',(1.,0.,0.));
#4970=DIRECTION('center_axis',(0.,0.,1.));
#4971=DIRECTION('ref_axis',(1.,0.,0.));
#4972=DIRECTION('center_axis',(0.,0.,1.));
#4973=DIRECTION('ref_axis',(1.,0.,0.));
#4974=DIRECTION('',(0.,0.,1.));
#4975=DIRECTION('center_axis',(0.,0.,-1.));
#4976=DIRECTION('ref_axis',(1.,0.,0.));
#4977=DIRECTION('center_axis',(0.,1.,0.));
#4978=DIRECTION('ref_axis',(-1.,0.,0.));
#4979=DIRECTION('',(-1.,0.,0.));
#4980=DIRECTION('',(0.,0.,1.));
#4981=DIRECTION('',(-1.,0.,0.));
#4982=DIRECTION('',(0.,0.,1.));
#4983=DIRECTION('center_axis',(1.,0.,0.));
#4984=DIRECTION('ref_axis',(0.,1.,0.));
#4985=DIRECTION('',(0.,1.,0.));
#4986=DIRECTION('',(0.,1.,0.));
#4987=DIRECTION('',(0.,0.,1.));
#4988=DIRECTION('center_axis',(0.,-1.,0.));
#4989=DIRECTION('ref_axis',(1.,0.,0.));
#4990=DIRECTION('',(1.,0.,0.));
#4991=DIRECTION('',(1.,0.,0.));
#4992=DIRECTION('',(0.,0.,1.));
#4993=DIRECTION('center_axis',(-1.,0.,0.));
#4994=DIRECTION('ref_axis',(0.,-1.,0.));
#4995=DIRECTION('',(0.,-1.,0.));
#4996=DIRECTION('',(0.,-1.,0.));
#4997=DIRECTION('center_axis',(0.,0.,1.));
#4998=DIRECTION('ref_axis',(1.,0.,0.));
#4999=DIRECTION('center_axis',(0.,0.,1.));
#5000=DIRECTION('ref_axis',(1.,0.,0.));
#6088=CARTESIAN_POINT('',(0.,0.,0.));
#6089=CARTESIAN_POINT('Origin',(12.5,-0.3,0.7));
#6090=CARTESIAN_POINT('',(14.5,-0.3,1.));
#6091=CARTESIAN_POINT('',(12.5,-0.3,1.));
#6092=CARTESIAN_POINT('',(11.25,-0.3,1.));
#6093=CARTESIAN_POINT('',(14.5,-0.3,0.7));
#6094=CARTESIAN_POINT('',(14.5,-0.3,0.7));
#6095=CARTESIAN_POINT('',(12.5,-0.3,0.7));
#6096=CARTESIAN_POINT('',(12.5,-0.3,0.7));
#6097=CARTESIAN_POINT('',(12.5,-0.3,0.7));
#6098=CARTESIAN_POINT('Origin',(12.5,0.3,0.7));
#6099=CARTESIAN_POINT('',(12.5,0.3,1.));
#6100=CARTESIAN_POINT('',(12.5,0.15,1.));
#6101=CARTESIAN_POINT('',(12.5,0.3,0.7));
#6102=CARTESIAN_POINT('',(12.5,0.3,0.7));
#6103=CARTESIAN_POINT('',(12.5,0.3,0.7));
#6104=CARTESIAN_POINT('Origin',(14.5,0.3,0.7));
#6105=CARTESIAN_POINT('',(14.5,0.3,1.));
#6106=CARTESIAN_POINT('',(12.25,0.3,1.));
#6107=CARTESIAN_POINT('',(14.5,0.3,0.7));
#6108=CARTESIAN_POINT('',(14.5,0.3,0.7));
#6109=CARTESIAN_POINT('',(14.5,0.3,0.7));
#6110=CARTESIAN_POINT('Origin',(14.5,-0.3,0.7));
#6111=CARTESIAN_POINT('',(14.5,-0.15,1.));
#6112=CARTESIAN_POINT('',(14.5,-0.3,0.7));
#6113=CARTESIAN_POINT('Origin',(13.5,0.,0.7));
#6114=CARTESIAN_POINT('Origin',(5.5,-0.3,0.7));
#6115=CARTESIAN_POINT('',(7.5,-0.3,1.));
#6116=CARTESIAN_POINT('',(5.5,-0.3,1.));
#6117=CARTESIAN_POINT('',(7.75,-0.3,1.));
#6118=CARTESIAN_POINT('',(7.5,-0.3,0.7));
#6119=CARTESIAN_POINT('',(7.5,-0.3,0.7));
#6120=CARTESIAN_POINT('',(5.5,-0.3,0.7));
#6121=CARTESIAN_POINT('',(5.5,-0.3,0.7));
#6122=CARTESIAN_POINT('',(5.5,-0.3,0.7));
#6123=CARTESIAN_POINT('Origin',(5.5,0.3,0.7));
#6124=CARTESIAN_POINT('',(5.5,0.3,1.));
#6125=CARTESIAN_POINT('',(5.5,0.15,1.));
#6126=CARTESIAN_POINT('',(5.5,0.3,0.7));
#6127=CARTESIAN_POINT('',(5.5,0.3,0.7));
#6128=CARTESIAN_POINT('',(5.5,0.3,0.7));
#6129=CARTESIAN_POINT('Origin',(7.5,0.3,0.7));
#6130=CARTESIAN_POINT('',(7.5,0.3,1.));
#6131=CARTESIAN_POINT('',(8.75,0.3,1.));
#6132=CARTESIAN_POINT('',(7.5,0.3,0.7));
#6133=CARTESIAN_POINT('',(7.5,0.3,0.7));
#6134=CARTESIAN_POINT('',(7.5,0.3,0.7));
#6135=CARTESIAN_POINT('Origin',(7.5,-0.3,0.7));
#6136=CARTESIAN_POINT('',(7.5,-0.15,1.));
#6137=CARTESIAN_POINT('',(7.5,-0.3,0.7));
#6138=CARTESIAN_POINT('Origin',(6.5,0.,0.7));
#6139=CARTESIAN_POINT('Origin',(17.,-4.5,-0.1));
#6140=CARTESIAN_POINT('',(16.725,-4.5,0.));
#6141=CARTESIAN_POINT('Origin',(17.,-4.5,0.));
#6142=CARTESIAN_POINT('',(16.725,-4.5,1.));
#6143=CARTESIAN_POINT('',(16.725,-4.5,-0.1));
#6144=CARTESIAN_POINT('Origin',(17.,-4.5,1.));
#6145=CARTESIAN_POINT('Origin',(3.,4.5,-0.1));
#6146=CARTESIAN_POINT('',(2.725,4.5,0.));
#6147=CARTESIAN_POINT('Origin',(3.,4.5,0.));
#6148=CARTESIAN_POINT('',(2.725,4.5,1.));
#6149=CARTESIAN_POINT('',(2.725,4.5,-0.1));
#6150=CARTESIAN_POINT('Origin',(3.,4.5,1.));
#6151=CARTESIAN_POINT('Origin',(3.,-4.5,-0.1));
#6152=CARTESIAN_POINT('',(2.725,-4.5,0.));
#6153=CARTESIAN_POINT('Origin',(3.,-4.5,0.));
#6154=CARTESIAN_POINT('',(2.725,-4.5,1.));
#6155=CARTESIAN_POINT('',(2.725,-4.5,-0.1));
#6156=CARTESIAN_POINT('Origin',(3.,-4.5,1.));
#6157=CARTESIAN_POINT('Origin',(17.,4.5,-0.1));
#6158=CARTESIAN_POINT('',(16.725,4.5,0.));
#6159=CARTESIAN_POINT('Origin',(17.,4.5,0.));
#6160=CARTESIAN_POINT('',(16.725,4.5,1.));
#6161=CARTESIAN_POINT('',(16.725,4.5,-0.1));
#6162=CARTESIAN_POINT('Origin',(17.,4.5,1.));
#6163=CARTESIAN_POINT('Origin',(10.,-4.,-0.1));
#6164=CARTESIAN_POINT('',(9.66,-4.,0.));
#6165=CARTESIAN_POINT('Origin',(10.,-4.,0.));
#6166=CARTESIAN_POINT('',(9.66,-4.,1.));
#6167=CARTESIAN_POINT('',(9.66,-4.,-0.1));
#6168=CARTESIAN_POINT('Origin',(10.,-4.,1.));
#6169=CARTESIAN_POINT('Origin',(10.,4.,-0.1));
#6170=CARTESIAN_POINT('',(9.66,4.,0.));
#6171=CARTESIAN_POINT('Origin',(10.,4.,0.));
#6172=CARTESIAN_POINT('',(9.66,4.,1.));
#6173=CARTESIAN_POINT('',(9.66,4.,-0.1));
#6174=CARTESIAN_POINT('Origin',(10.,4.,1.));
#6175=CARTESIAN_POINT('Origin',(2.,-1.4,-0.1));
#6176=CARTESIAN_POINT('',(1.75,-1.4,0.));
#6177=CARTESIAN_POINT('Origin',(2.,-1.4,0.));
#6178=CARTESIAN_POINT('',(1.75,-1.4,1.));
#6179=CARTESIAN_POINT('',(1.75,-1.4,-0.1));
#6180=CARTESIAN_POINT('Origin',(2.,-1.4,1.));
#6181=CARTESIAN_POINT('Origin',(6.5,-2.5,-0.1));
#6182=CARTESIAN_POINT('',(6.25,-2.5,0.));
#6183=CARTESIAN_POINT('Origin',(6.5,-2.5,0.));
#6184=CARTESIAN_POINT('',(6.25,-2.5,1.));
#6185=CARTESIAN_POINT('',(6.25,-2.5,-0.1));
#6186=CARTESIAN_POINT('Origin',(6.5,-2.5,1.));
#6187=CARTESIAN_POINT('Origin',(6.5,2.5,-0.1));
#6188=CARTESIAN_POINT('',(6.25,2.5,0.));
#6189=CARTESIAN_POINT('Origin',(6.5,2.5,0.));
#6190=CARTESIAN_POINT('',(6.25,2.5,1.));
#6191=CARTESIAN_POINT('',(6.25,2.5,-0.1));
#6192=CARTESIAN_POINT('Origin',(6.5,2.5,1.));
#6193=CARTESIAN_POINT('Origin',(13.5,-2.5,-0.1));
#6194=CARTESIAN_POINT('',(13.25,-2.5,0.));
#6195=CARTESIAN_POINT('Origin',(13.5,-2.5,0.));
#6196=CARTESIAN_POINT('',(13.25,-2.5,1.));
#6197=CARTESIAN_POINT('',(13.25,-2.5,-0.1));
#6198=CARTESIAN_POINT('Origin',(13.5,-2.5,1.));
#6199=CARTESIAN_POINT('Origin',(13.5,2.5,-0.1));
#6200=CARTESIAN_POINT('',(13.25,2.5,0.));
#6201=CARTESIAN_POINT('Origin',(13.5,2.5,0.));
#6202=CARTESIAN_POINT('',(13.25,2.5,1.));
#6203=CARTESIAN_POINT('',(13.25,2.5,-0.1));
#6204=CARTESIAN_POINT('Origin',(13.5,2.5,1.));
#6205=CARTESIAN_POINT('Origin',(2.,1.4,-0.1));
#6206=CARTESIAN_POINT('',(1.75,1.4,0.));
#6207=CARTESIAN_POINT('Origin',(2.,1.4,0.));
#6208=CARTESIAN_POINT('',(1.75,1.4,1.));
#6209=CARTESIAN_POINT('',(1.75,1.4,-0.1));
#6210=CARTESIAN_POINT('Origin',(2.,1.4,1.));
#6211=CARTESIAN_POINT('Origin',(20.,5.5,0.));
#6212=CARTESIAN_POINT('',(20.,5.5,0.));
#6213=CARTESIAN_POINT('',(0.,5.5,0.));
#6214=CARTESIAN_POINT('',(20.,5.5,0.));
#6215=CARTESIAN_POINT('',(0.,5.5,1.));
#6216=CARTESIAN_POINT('',(0.,5.5,0.));
#6217=CARTESIAN_POINT('',(20.,5.5,1.));
#6218=CARTESIAN_POINT('',(20.,5.5,1.));
#6219=CARTESIAN_POINT('',(20.,5.5,0.));
#6220=CARTESIAN_POINT('Origin',(20.,-5.5,0.));
#6221=CARTESIAN_POINT('',(20.,-5.5,0.));
#6222=CARTESIAN_POINT('',(20.,-5.5,0.));
#6223=CARTESIAN_POINT('',(20.,-5.5,1.));
#6224=CARTESIAN_POINT('',(20.,-5.5,1.));
#6225=CARTESIAN_POINT('',(20.,-5.5,0.));
#6226=CARTESIAN_POINT('Origin',(0.,-5.5,0.));
#6227=CARTESIAN_POINT('',(0.,-5.5,0.));
#6228=CARTESIAN_POINT('',(0.,-5.5,0.));
#6229=CARTESIAN_POINT('',(0.,-5.5,1.));
#6230=CARTESIAN_POINT('',(0.,-5.5,1.));
#6231=CARTESIAN_POINT('',(0.,-5.5,0.));
#6232=CARTESIAN_POINT('Origin',(0.,5.5,0.));
#6233=CARTESIAN_POINT('',(0.,5.5,0.));
#6234=CARTESIAN_POINT('',(0.,5.5,1.));
#6235=CARTESIAN_POINT('Origin',(10.,0.,1.));
#6236=CARTESIAN_POINT('Origin',(10.,0.,0.));
#7295=UNCERTAINTY_MEASURE_WITH_UNIT(LENGTH_MEASURE(0.001),#7345,
'DISTANCE_ACCURACY_VALUE',
'Maximum model space distance between geometric entities at asserted c
onnectivities');
#7318=UNCERTAINTY_MEASURE_WITH_UNIT(LENGTH_MEASURE(0.001),#7345,
'DISTANCE_ACCURACY_VALUE',
'Maximum model space distance between geometric entities at asserted c
onnectivities');
#7321=(
GEOMETRIC_REPRESENTATION_CONTEXT(3)
GLOBAL_UNCERTAINTY_ASSIGNED_CONTEXT((#7295))
GLOBAL_UNIT_ASSIGNED_CONTEXT((#7345,#7347,#7348))
REPRESENTATION_CONTEXT('','3D')
);
#7344=(
GEOMETRIC_REPRESENTATION_CONTEXT(3)
GLOBAL_UNCERTAINTY_ASSIGNED_CONTEXT((#7318))
GLOBAL_UNIT_ASSIGNED_CONTEXT((#7345,#7347,#7348))
REPRESENTATION_CONTEXT('','3D')
);
#7345=(
LENGTH_UNIT()
NAMED_UNIT(*)
SI_UNIT(.CENTI.,.METRE.)
);
#7347=(
NAMED_UNIT(*)
PLANE_ANGLE_UNIT()
SI_UNIT($,.RADIAN.)
);
#7348=(
NAMED_UNIT(*)
SI_UNIT($,.STERADIAN.)
SOLID_ANGLE_UNIT()
);
#7351=SHAPE_DEFINITION_REPRESENTATION(#7376,#7442);
#7376=PRODUCT_DEFINITION_SHAPE('',$,#7468);
#7442=SHAPE_REPRESENTATION('',(#4406),#7321);
#7465=PRODUCT_DEFINITION_CONTEXT('part definition',#7542,'design');
#7468=PRODUCT_DEFINITION('Base','Base',#7493,#7465);
#7493=PRODUCT_DEFINITION_FORMATION('',$,#7546);
#7542=APPLICATION_CONTEXT(
'Core Data for Automotive Mechanical Design Process');
#7543=PRODUCT_CONTEXT('part definition',#7542,'mechanical');
#7546=PRODUCT('Base','Base','Base',(#7543));
#7604=COLOUR_RGB('Dark Blue',0.08,0.2,0.34);
#7605=FILL_AREA_STYLE_COLOUR('',#7604);
#7606=FILL_AREA_STYLE('',(#7605));
#7607=SURFACE_STYLE_FILL_AREA(#7606);
#7608=SURFACE_SIDE_STYLE('',(#7607));
#7609=SURFACE_STYLE_USAGE(.BOTH.,#7608);
#7610=PRESENTATION_STYLE_ASSIGNMENT((#7609));
ENDSEC;
END-ISO-10303-21;
